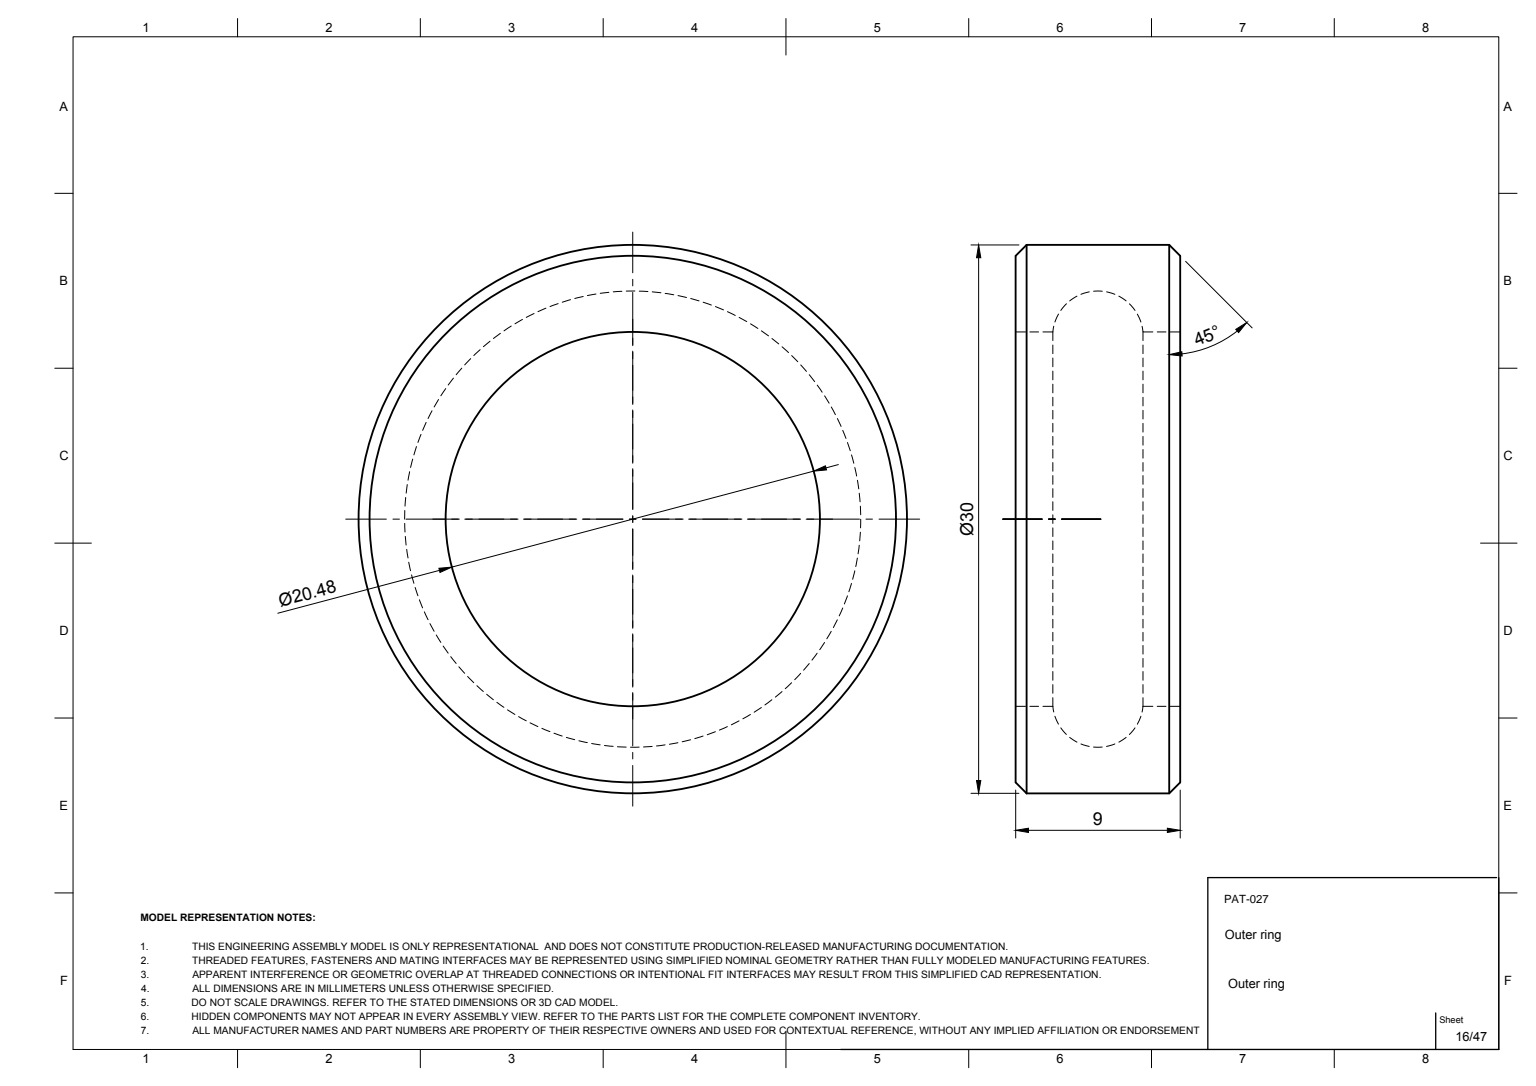
ISO-10303-21;
HEADER;
/* Generated by software containing ST-Developer
 * from STEP Tools, Inc. (www.steptools.com) 
 */

FILE_DESCRIPTION(
/* description */ ('Crank-driven oscillating fan base (mechanism only)'),

/* implementation_level */ '2;1');

FILE_NAME(
/* name */ 'Outer ring.step',
/* time_stamp */ '2026-10-28T03:25:00-07:00',
/* author */ (''),
/* organization */ (''),
/* preprocessor_version */ 'ST-DEVELOPER v20.2',
/* originating_system */ 'Autodesk Translation Framework v15.17.0.0',
/* authorisation */ '');

FILE_SCHEMA (('AUTOMOTIVE_DESIGN { 1 0 10303 214 3 1 1 }'));
ENDSEC;

DATA;
#10=MECHANICAL_DESIGN_GEOMETRIC_PRESENTATION_REPRESENTATION('',(#447),#11916);
#292=TOROIDAL_SURFACE('',#6851,1.,0.247676);
#298=CONICAL_SURFACE('',#6862,1.47,0.785398163397449);
#299=CONICAL_SURFACE('',#6866,1.47,0.785398163397449);
#367=SHAPE_REPRESENTATION_RELATIONSHIP('SRR','None',#12092,#407);
#407=ADVANCED_BREP_SHAPE_REPRESENTATION('',(#494),#11883);
#447=STYLED_ITEM('',(#12375),#494);
#494=MANIFOLD_SOLID_BREP('Body1',#6078);
#609=FACE_BOUND('',#1475,.T.);
#610=FACE_BOUND('',#1480,.T.);
#755=PLANE('',#6859);
#756=PLANE('',#6868);
#1018=FACE_OUTER_BOUND('',#1472,.T.);
#1019=FACE_OUTER_BOUND('',#1473,.T.);
#1020=FACE_OUTER_BOUND('',#1474,.T.);
#1021=FACE_OUTER_BOUND('',#1476,.T.);
#1022=FACE_OUTER_BOUND('',#1477,.T.);
#1023=FACE_OUTER_BOUND('',#1478,.T.);
#1024=FACE_OUTER_BOUND('',#1479,.T.);
#1025=FACE_OUTER_BOUND('',#1481,.T.);
#1472=EDGE_LOOP('',(#4636,#4637,#4638,#4639,#4640,#4641));
#1473=EDGE_LOOP('',(#4642,#4643,#4644,#4645,#4646));
#1474=EDGE_LOOP('',(#4647));
#1475=EDGE_LOOP('',(#4648));
#1476=EDGE_LOOP('',(#4649,#4650,#4651,#4652));
#1477=EDGE_LOOP('',(#4653,#4654,#4655,#4656));
#1478=EDGE_LOOP('',(#4657,#4658,#4659,#4660));
#1479=EDGE_LOOP('',(#4661));
#1480=EDGE_LOOP('',(#4662));
#1481=EDGE_LOOP('',(#4663,#4664,#4665,#4666,#4667));
#1928=LINE('',#10216,#2261);
#1929=LINE('',#10225,#2262);
#1930=LINE('',#10229,#2263);
#1931=LINE('',#10233,#2264);
#1932=LINE('',#10236,#2265);
#2261=VECTOR('',#8141,1.023815);
#2262=VECTOR('',#8152,1.47);
#2263=VECTOR('',#8157,1.5);
#2264=VECTOR('',#8162,1.47);
#2265=VECTOR('',#8167,1.023815);
#2610=CIRCLE('',#6852,1.023815);
#2611=CIRCLE('',#6853,1.023815);
#2612=CIRCLE('',#6854,0.247676);
#2613=CIRCLE('',#6855,1.023815);
#2614=CIRCLE('',#6856,1.023815);
#2615=CIRCLE('',#6858,1.023815);
#2616=CIRCLE('',#6860,1.44);
#2617=CIRCLE('',#6861,1.023815);
#2618=CIRCLE('',#6863,1.5);
#2619=CIRCLE('',#6865,1.5);
#2620=CIRCLE('',#6867,1.44);
#3018=VERTEX_POINT('',#10204);
#3019=VERTEX_POINT('',#10205);
#3020=VERTEX_POINT('',#10208);
#3021=VERTEX_POINT('',#10210);
#3022=VERTEX_POINT('',#10214);
#3023=VERTEX_POINT('',#10218);
#3024=VERTEX_POINT('',#10220);
#3025=VERTEX_POINT('',#10223);
#3026=VERTEX_POINT('',#10227);
#3027=VERTEX_POINT('',#10231);
#3613=EDGE_CURVE('',#3018,#3019,#2610,.T.);
#3614=EDGE_CURVE('',#3019,#3018,#2611,.T.);
#3615=EDGE_CURVE('',#3019,#3020,#2612,.T.);
#3616=EDGE_CURVE('',#3021,#3020,#2613,.T.);
#3617=EDGE_CURVE('',#3020,#3021,#2614,.T.);
#3618=EDGE_CURVE('',#3022,#3022,#2615,.T.);
#3619=EDGE_CURVE('',#3022,#3021,#1928,.T.);
#3620=EDGE_CURVE('',#3023,#3023,#2616,.T.);
#3621=EDGE_CURVE('',#3024,#3024,#2617,.T.);
#3622=EDGE_CURVE('',#3025,#3025,#2618,.T.);
#3623=EDGE_CURVE('',#3025,#3023,#1929,.T.);
#3624=EDGE_CURVE('',#3026,#3026,#2619,.T.);
#3625=EDGE_CURVE('',#3026,#3025,#1930,.T.);
#3626=EDGE_CURVE('',#3027,#3027,#2620,.T.);
#3627=EDGE_CURVE('',#3027,#3026,#1931,.T.);
#3628=EDGE_CURVE('',#3018,#3024,#1932,.T.);
#4636=ORIENTED_EDGE('',*,*,#3613,.F.);
#4637=ORIENTED_EDGE('',*,*,#3614,.F.);
#4638=ORIENTED_EDGE('',*,*,#3615,.T.);
#4639=ORIENTED_EDGE('',*,*,#3616,.F.);
#4640=ORIENTED_EDGE('',*,*,#3617,.F.);
#4641=ORIENTED_EDGE('',*,*,#3615,.F.);
#4642=ORIENTED_EDGE('',*,*,#3618,.T.);
#4643=ORIENTED_EDGE('',*,*,#3619,.T.);
#4644=ORIENTED_EDGE('',*,*,#3616,.T.);
#4645=ORIENTED_EDGE('',*,*,#3617,.T.);
#4646=ORIENTED_EDGE('',*,*,#3619,.F.);
#4647=ORIENTED_EDGE('',*,*,#3620,.F.);
#4648=ORIENTED_EDGE('',*,*,#3621,.T.);
#4649=ORIENTED_EDGE('',*,*,#3622,.F.);
#4650=ORIENTED_EDGE('',*,*,#3623,.T.);
#4651=ORIENTED_EDGE('',*,*,#3620,.T.);
#4652=ORIENTED_EDGE('',*,*,#3623,.F.);
#4653=ORIENTED_EDGE('',*,*,#3624,.F.);
#4654=ORIENTED_EDGE('',*,*,#3625,.T.);
#4655=ORIENTED_EDGE('',*,*,#3622,.T.);
#4656=ORIENTED_EDGE('',*,*,#3625,.F.);
#4657=ORIENTED_EDGE('',*,*,#3626,.F.);
#4658=ORIENTED_EDGE('',*,*,#3627,.T.);
#4659=ORIENTED_EDGE('',*,*,#3624,.T.);
#4660=ORIENTED_EDGE('',*,*,#3627,.F.);
#4661=ORIENTED_EDGE('',*,*,#3626,.T.);
#4662=ORIENTED_EDGE('',*,*,#3618,.F.);
#4663=ORIENTED_EDGE('',*,*,#3613,.T.);
#4664=ORIENTED_EDGE('',*,*,#3614,.T.);
#4665=ORIENTED_EDGE('',*,*,#3628,.T.);
#4666=ORIENTED_EDGE('',*,*,#3621,.F.);
#4667=ORIENTED_EDGE('',*,*,#3628,.F.);
#5609=CYLINDRICAL_SURFACE('',#6857,1.023815);
#5610=CYLINDRICAL_SURFACE('',#6864,1.5);
#5611=CYLINDRICAL_SURFACE('',#6869,1.023815);
#5824=ADVANCED_FACE('',(#1018),#292,.F.);
#5825=ADVANCED_FACE('',(#1019),#5609,.F.);
#5826=ADVANCED_FACE('',(#1020,#609),#755,.T.);
#5827=ADVANCED_FACE('',(#1021),#298,.T.);
#5828=ADVANCED_FACE('',(#1022),#5610,.T.);
#5829=ADVANCED_FACE('',(#1023),#299,.T.);
#5830=ADVANCED_FACE('',(#1024,#610),#756,.T.);
#5831=ADVANCED_FACE('',(#1025),#5611,.F.);
#6078=CLOSED_SHELL('',(#5824,#5825,#5826,#5827,#5828,#5829,#5830,#5831));
#6850=AXIS2_PLACEMENT_3D('',#10202,#8123,#8124);
#6851=AXIS2_PLACEMENT_3D('',#10203,#8125,#8126);
#6852=AXIS2_PLACEMENT_3D('',#10206,#8127,#8128);
#6853=AXIS2_PLACEMENT_3D('',#10207,#8129,#8130);
#6854=AXIS2_PLACEMENT_3D('',#10209,#8131,#8132);
#6855=AXIS2_PLACEMENT_3D('',#10211,#8133,#8134);
#6856=AXIS2_PLACEMENT_3D('',#10212,#8135,#8136);
#6857=AXIS2_PLACEMENT_3D('',#10213,#8137,#8138);
#6858=AXIS2_PLACEMENT_3D('',#10215,#8139,#8140);
#6859=AXIS2_PLACEMENT_3D('',#10217,#8142,#8143);
#6860=AXIS2_PLACEMENT_3D('',#10219,#8144,#8145);
#6861=AXIS2_PLACEMENT_3D('',#10221,#8146,#8147);
#6862=AXIS2_PLACEMENT_3D('',#10222,#8148,#8149);
#6863=AXIS2_PLACEMENT_3D('',#10224,#8150,#8151);
#6864=AXIS2_PLACEMENT_3D('',#10226,#8153,#8154);
#6865=AXIS2_PLACEMENT_3D('',#10228,#8155,#8156);
#6866=AXIS2_PLACEMENT_3D('',#10230,#8158,#8159);
#6867=AXIS2_PLACEMENT_3D('',#10232,#8160,#8161);
#6868=AXIS2_PLACEMENT_3D('',#10234,#8163,#8164);
#6869=AXIS2_PLACEMENT_3D('',#10235,#8165,#8166);
#8123=DIRECTION('axis',(0.,0.,1.));
#8124=DIRECTION('refdir',(1.,0.,0.));
#8125=DIRECTION('center_axis',(0.,-1.,0.));
#8126=DIRECTION('ref_axis',(0.,0.,-1.));
#8127=DIRECTION('center_axis',(0.,-1.,0.));
#8128=DIRECTION('ref_axis',(1.,0.,0.));
#8129=DIRECTION('center_axis',(0.,-1.,0.));
#8130=DIRECTION('ref_axis',(1.,0.,0.));
#8131=DIRECTION('center_axis',(1.,0.,1.22464679914735E-16));
#8132=DIRECTION('ref_axis',(-1.22464679914735E-16,0.,1.));
#8133=DIRECTION('center_axis',(0.,1.,0.));
#8134=DIRECTION('ref_axis',(1.,0.,0.));
#8135=DIRECTION('center_axis',(0.,1.,0.));
#8136=DIRECTION('ref_axis',(1.,0.,0.));
#8137=DIRECTION('center_axis',(0.,-1.,0.));
#8138=DIRECTION('ref_axis',(1.,0.,0.));
#8139=DIRECTION('center_axis',(0.,-1.,0.));
#8140=DIRECTION('ref_axis',(1.,0.,0.));
#8141=DIRECTION('',(0.,1.,0.));
#8142=DIRECTION('center_axis',(0.,1.,0.));
#8143=DIRECTION('ref_axis',(0.,0.,1.));
#8144=DIRECTION('center_axis',(0.,-1.,0.));
#8145=DIRECTION('ref_axis',(1.,0.,0.));
#8146=DIRECTION('center_axis',(0.,-1.,0.));
#8147=DIRECTION('ref_axis',(1.,0.,0.));
#8148=DIRECTION('center_axis',(0.,-1.,0.));
#8149=DIRECTION('ref_axis',(1.,0.,0.));
#8150=DIRECTION('center_axis',(0.,-1.,0.));
#8151=DIRECTION('ref_axis',(1.,0.,0.));
#8152=DIRECTION('',(0.707106781186548,0.707106781186547,8.65956056235494E-17));
#8153=DIRECTION('center_axis',(0.,-1.,0.));
#8154=DIRECTION('ref_axis',(1.,0.,0.));
#8155=DIRECTION('center_axis',(0.,-1.,0.));
#8156=DIRECTION('ref_axis',(1.,0.,0.));
#8157=DIRECTION('',(0.,1.,0.));
#8158=DIRECTION('center_axis',(0.,1.,0.));
#8159=DIRECTION('ref_axis',(1.,0.,0.));
#8160=DIRECTION('center_axis',(0.,-1.,0.));
#8161=DIRECTION('ref_axis',(1.,0.,0.));
#8162=DIRECTION('',(-0.707106781186548,0.707106781186547,-8.65956056235494E-17));
#8163=DIRECTION('center_axis',(0.,-1.,0.));
#8164=DIRECTION('ref_axis',(0.,0.,-1.));
#8165=DIRECTION('center_axis',(0.,-1.,0.));
#8166=DIRECTION('ref_axis',(1.,0.,0.));
#8167=DIRECTION('',(0.,1.,0.));
#10202=CARTESIAN_POINT('',(0.,0.,0.));
#10203=CARTESIAN_POINT('Origin',(0.,0.,0.));
#10204=CARTESIAN_POINT('',(-1.023815,0.246528389340863,-1.25381176266905E-16));
#10205=CARTESIAN_POINT('',(-1.25381176266905E-16,0.246528389340863,1.023815));
#10206=CARTESIAN_POINT('Origin',(0.,0.246528389340863,0.));
#10207=CARTESIAN_POINT('Origin',(0.,0.246528389340863,0.));
#10208=CARTESIAN_POINT('',(-1.25381176266905E-16,-0.246528389340863,1.023815));
#10209=CARTESIAN_POINT('Origin',(-1.22464679914735E-16,0.,1.));
#10210=CARTESIAN_POINT('',(-1.023815,-0.246528389340863,1.25381176266905E-16));
#10211=CARTESIAN_POINT('Origin',(0.,-0.246528389340863,0.));
#10212=CARTESIAN_POINT('Origin',(0.,-0.246528389340863,0.));
#10213=CARTESIAN_POINT('Origin',(0.,0.,0.));
#10214=CARTESIAN_POINT('',(-1.023815,-0.45,-1.25381176266905E-16));
#10215=CARTESIAN_POINT('Origin',(0.,-0.45,0.));
#10216=CARTESIAN_POINT('',(-1.023815,0.,-1.25381176266905E-16));
#10217=CARTESIAN_POINT('Origin',(1.44,0.45,0.));
#10218=CARTESIAN_POINT('',(-1.44,0.45,-1.76349139077219E-16));
#10219=CARTESIAN_POINT('Origin',(0.,0.45,0.));
#10220=CARTESIAN_POINT('',(-1.023815,0.45,-1.25381176266905E-16));
#10221=CARTESIAN_POINT('Origin',(0.,0.45,0.));
#10222=CARTESIAN_POINT('Origin',(0.,0.42,0.));
#10223=CARTESIAN_POINT('',(-1.5,0.39,-1.83697019872103E-16));
#10224=CARTESIAN_POINT('Origin',(0.,0.39,0.));
#10225=CARTESIAN_POINT('',(-1.47,0.42,-1.80023079474661E-16));
#10226=CARTESIAN_POINT('Origin',(0.,0.,0.));
#10227=CARTESIAN_POINT('',(-1.5,-0.39,-1.83697019872103E-16));
#10228=CARTESIAN_POINT('Origin',(0.,-0.39,0.));
#10229=CARTESIAN_POINT('',(-1.5,0.,-1.83697019872103E-16));
#10230=CARTESIAN_POINT('Origin',(0.,-0.42,0.));
#10231=CARTESIAN_POINT('',(-1.44,-0.45,-1.76349139077219E-16));
#10232=CARTESIAN_POINT('Origin',(0.,-0.45,0.));
#10233=CARTESIAN_POINT('',(-1.47,-0.42,-1.80023079474661E-16));
#10234=CARTESIAN_POINT('Origin',(1.023815,-0.45,0.));
#10235=CARTESIAN_POINT('Origin',(0.,0.,0.));
#10236=CARTESIAN_POINT('',(-1.023815,0.,-1.25381176266905E-16));
#11836=UNCERTAINTY_MEASURE_WITH_UNIT(LENGTH_MEASURE(0.001),#11917,
'DISTANCE_ACCURACY_VALUE',
'Maximum model space distance between geometric entities at asserted c
onnectivities');
#11869=UNCERTAINTY_MEASURE_WITH_UNIT(LENGTH_MEASURE(0.001),#11917,
'DISTANCE_ACCURACY_VALUE',
'Maximum model space distance between geometric entities at asserted c
onnectivities');
#11883=(
GEOMETRIC_REPRESENTATION_CONTEXT(3)
GLOBAL_UNCERTAINTY_ASSIGNED_CONTEXT((#11836))
GLOBAL_UNIT_ASSIGNED_CONTEXT((#11917,#11919,#11920))
REPRESENTATION_CONTEXT('','3D')
);
#11916=(
GEOMETRIC_REPRESENTATION_CONTEXT(3)
GLOBAL_UNCERTAINTY_ASSIGNED_CONTEXT((#11869))
GLOBAL_UNIT_ASSIGNED_CONTEXT((#11917,#11919,#11920))
REPRESENTATION_CONTEXT('','3D')
);
#11917=(
LENGTH_UNIT()
NAMED_UNIT(*)
SI_UNIT(.CENTI.,.METRE.)
);
#11919=(
NAMED_UNIT(*)
PLANE_ANGLE_UNIT()
SI_UNIT($,.RADIAN.)
);
#11920=(
NAMED_UNIT(*)
SI_UNIT($,.STERADIAN.)
SOLID_ANGLE_UNIT()
);
#11934=SHAPE_DEFINITION_REPRESENTATION(#11980,#12092);
#11980=PRODUCT_DEFINITION_SHAPE('',$,#12139);
#12092=SHAPE_REPRESENTATION('',(#6850),#11883);
#12125=PRODUCT_DEFINITION_CONTEXT('part definition',#12265,'design');
#12139=PRODUCT_DEFINITION('Outer ring','Outer ring',#12185,#12125);
#12185=PRODUCT_DEFINITION_FORMATION('',$,#12280);
#12265=APPLICATION_CONTEXT(
'Core Data for Automotive Mechanical Design Process');
#12266=PRODUCT_CONTEXT('part definition',#12265,'mechanical');
#12280=PRODUCT('Outer ring','Outer ring','Outer ring',(#12266));
#12369=COLOUR_RGB('Grey',0.48,0.52,0.57);
#12370=FILL_AREA_STYLE_COLOUR('',#12369);
#12371=FILL_AREA_STYLE('',(#12370));
#12372=SURFACE_STYLE_FILL_AREA(#12371);
#12373=SURFACE_SIDE_STYLE('',(#12372));
#12374=SURFACE_STYLE_USAGE(.BOTH.,#12373);
#12375=PRESENTATION_STYLE_ASSIGNMENT((#12374));
ENDSEC;
END-ISO-10303-21;
